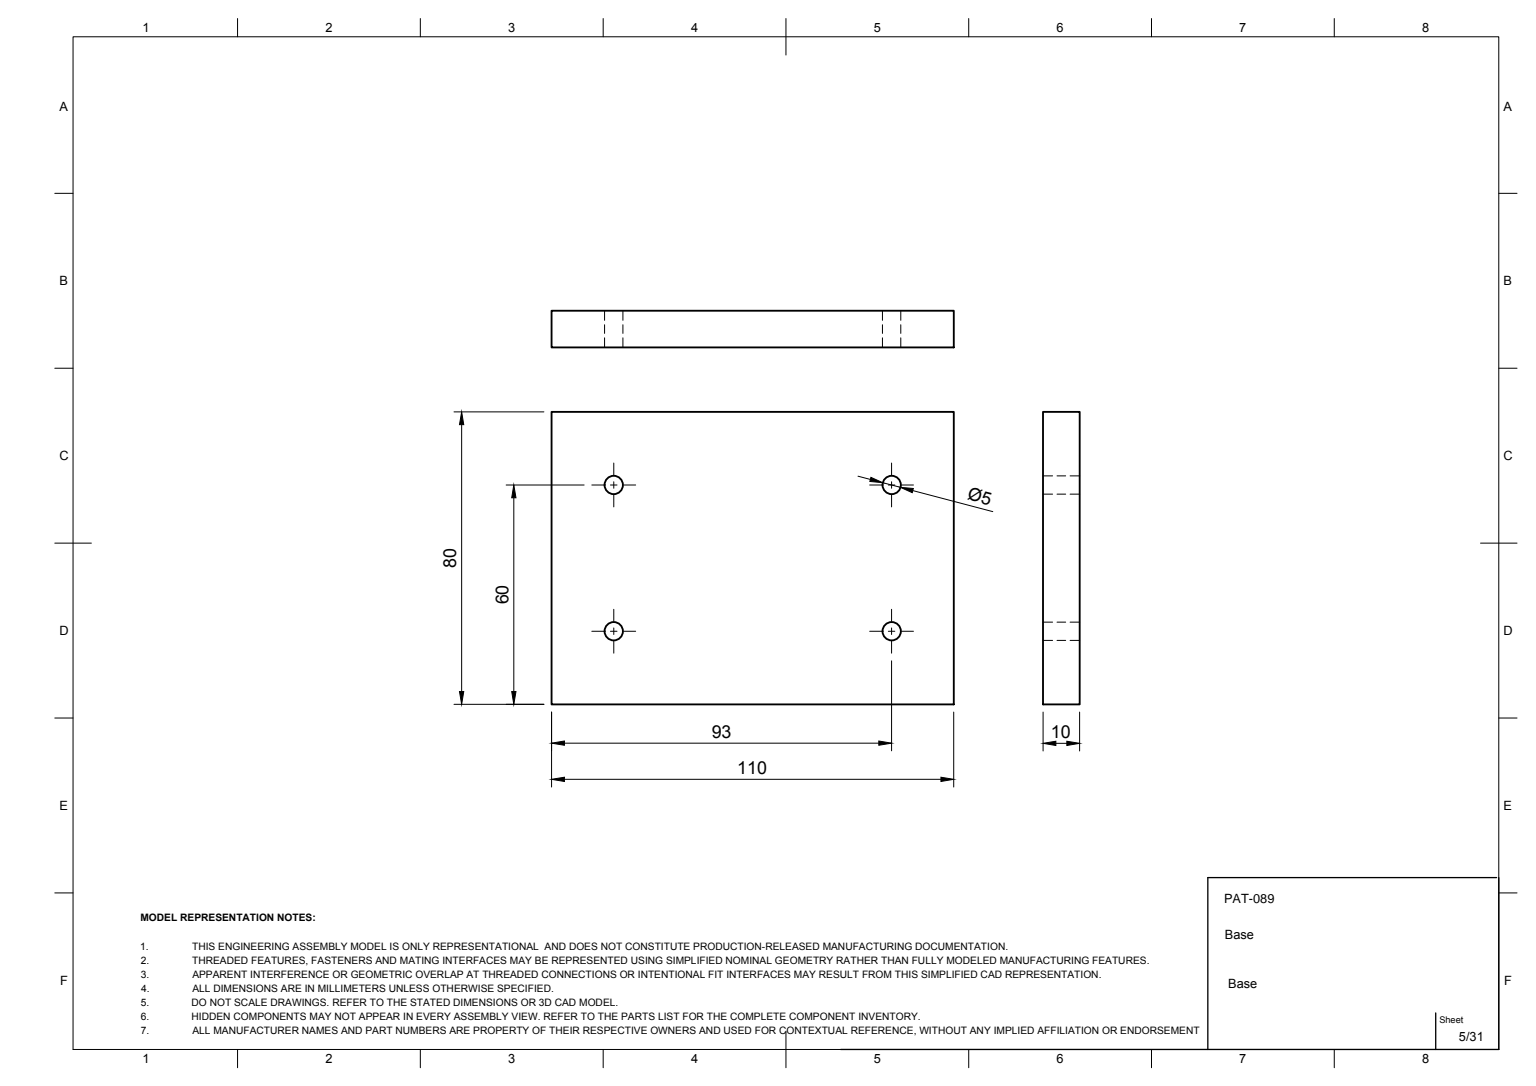
ISO-10303-21;
HEADER;
/* Generated by software containing ST-Developer
 * from STEP Tools, Inc. (www.steptools.com) 
 */

FILE_DESCRIPTION(
/* description */ ('Rotary union on bearing shaft'),
/* implementation_level */ '2;1');

FILE_NAME(
/* name */ 'Base.step',
/* time_stamp */ '2026-10-28T03:24:01-07:00',
/* author */ (''),
/* organization */ (''),
/* preprocessor_version */ 'ST-DEVELOPER v20.2',
/* originating_system */ 'Autodesk Translation Framework v15.17.0.0',
/* authorisation */ '');

FILE_SCHEMA (('AUTOMOTIVE_DESIGN { 1 0 10303 214 3 1 1 }'));
ENDSEC;

DATA;
#10=MECHANICAL_DESIGN_GEOMETRIC_PRESENTATION_REPRESENTATION('',(#313),#9448);
#259=SHAPE_REPRESENTATION_RELATIONSHIP('SRR','None',#9559,#286);
#286=ADVANCED_BREP_SHAPE_REPRESENTATION('',(#348),#9419);
#313=STYLED_ITEM('',(#9757),#348);
#348=MANIFOLD_SOLID_BREP('Body1',#4868);
#380=FACE_BOUND('',#964,.T.);
#381=FACE_BOUND('',#965,.T.);
#382=FACE_BOUND('',#966,.T.);
#383=FACE_BOUND('',#967,.T.);
#384=FACE_BOUND('',#969,.T.);
#385=FACE_BOUND('',#970,.T.);
#386=FACE_BOUND('',#971,.T.);
#387=FACE_BOUND('',#972,.T.);
#487=PLANE('',#5219);
#488=PLANE('',#5220);
#489=PLANE('',#5221);
#490=PLANE('',#5222);
#491=PLANE('',#5223);
#492=PLANE('',#5224);
#656=FACE_OUTER_BOUND('',#955,.T.);
#657=FACE_OUTER_BOUND('',#956,.T.);
#658=FACE_OUTER_BOUND('',#957,.T.);
#659=FACE_OUTER_BOUND('',#958,.T.);
#660=FACE_OUTER_BOUND('',#959,.T.);
#661=FACE_OUTER_BOUND('',#960,.T.);
#662=FACE_OUTER_BOUND('',#961,.T.);
#663=FACE_OUTER_BOUND('',#962,.T.);
#664=FACE_OUTER_BOUND('',#963,.T.);
#665=FACE_OUTER_BOUND('',#968,.T.);
#955=EDGE_LOOP('',(#3267,#3268,#3269,#3270));
#956=EDGE_LOOP('',(#3271,#3272,#3273,#3274));
#957=EDGE_LOOP('',(#3275,#3276,#3277,#3278));
#958=EDGE_LOOP('',(#3279,#3280,#3281,#3282));
#959=EDGE_LOOP('',(#3283,#3284,#3285,#3286));
#960=EDGE_LOOP('',(#3287,#3288,#3289,#3290));
#961=EDGE_LOOP('',(#3291,#3292,#3293,#3294));
#962=EDGE_LOOP('',(#3295,#3296,#3297,#3298));
#963=EDGE_LOOP('',(#3299,#3300,#3301,#3302));
#964=EDGE_LOOP('',(#3303));
#965=EDGE_LOOP('',(#3304));
#966=EDGE_LOOP('',(#3305));
#967=EDGE_LOOP('',(#3306));
#968=EDGE_LOOP('',(#3307,#3308,#3309,#3310));
#969=EDGE_LOOP('',(#3311));
#970=EDGE_LOOP('',(#3312));
#971=EDGE_LOOP('',(#3313));
#972=EDGE_LOOP('',(#3314));
#1361=LINE('',#7403,#1681);
#1362=LINE('',#7409,#1682);
#1363=LINE('',#7415,#1683);
#1364=LINE('',#7421,#1684);
#1365=LINE('',#7426,#1685);
#1366=LINE('',#7428,#1686);
#1367=LINE('',#7430,#1687);
#1368=LINE('',#7431,#1688);
#1369=LINE('',#7434,#1689);
#1370=LINE('',#7436,#1690);
#1371=LINE('',#7437,#1691);
#1372=LINE('',#7440,#1692);
#1373=LINE('',#7442,#1693);
#1374=LINE('',#7443,#1694);
#1375=LINE('',#7445,#1695);
#1376=LINE('',#7446,#1696);
#1681=VECTOR('',#5838,0.25);
#1682=VECTOR('',#5845,0.25);
#1683=VECTOR('',#5852,0.25);
#1684=VECTOR('',#5859,0.25);
#1685=VECTOR('',#5864,1.);
#1686=VECTOR('',#5865,1.);
#1687=VECTOR('',#5866,1.);
#1688=VECTOR('',#5867,1.);
#1689=VECTOR('',#5870,1.);
#1690=VECTOR('',#5871,1.);
#1691=VECTOR('',#5872,1.);
#1692=VECTOR('',#5875,1.);
#1693=VECTOR('',#5876,1.);
#1694=VECTOR('',#5877,1.);
#1695=VECTOR('',#5880,1.);
#1696=VECTOR('',#5881,1.);
#2001=CIRCLE('',#5208,0.25);
#2002=CIRCLE('',#5209,0.25);
#2003=CIRCLE('',#5211,0.25);
#2004=CIRCLE('',#5212,0.25);
#2005=CIRCLE('',#5214,0.25);
#2006=CIRCLE('',#5215,0.25);
#2007=CIRCLE('',#5217,0.25);
#2008=CIRCLE('',#5218,0.25);
#2253=VERTEX_POINT('',#7400);
#2254=VERTEX_POINT('',#7402);
#2255=VERTEX_POINT('',#7406);
#2256=VERTEX_POINT('',#7408);
#2257=VERTEX_POINT('',#7412);
#2258=VERTEX_POINT('',#7414);
#2259=VERTEX_POINT('',#7418);
#2260=VERTEX_POINT('',#7420);
#2261=VERTEX_POINT('',#7424);
#2262=VERTEX_POINT('',#7425);
#2263=VERTEX_POINT('',#7427);
#2264=VERTEX_POINT('',#7429);
#2265=VERTEX_POINT('',#7433);
#2266=VERTEX_POINT('',#7435);
#2267=VERTEX_POINT('',#7439);
#2268=VERTEX_POINT('',#7441);
#2661=EDGE_CURVE('',#2253,#2253,#2001,.T.);
#2662=EDGE_CURVE('',#2253,#2254,#1361,.T.);
#2663=EDGE_CURVE('',#2254,#2254,#2002,.T.);
#2664=EDGE_CURVE('',#2255,#2255,#2003,.T.);
#2665=EDGE_CURVE('',#2255,#2256,#1362,.T.);
#2666=EDGE_CURVE('',#2256,#2256,#2004,.T.);
#2667=EDGE_CURVE('',#2257,#2257,#2005,.T.);
#2668=EDGE_CURVE('',#2257,#2258,#1363,.T.);
#2669=EDGE_CURVE('',#2258,#2258,#2006,.T.);
#2670=EDGE_CURVE('',#2259,#2259,#2007,.T.);
#2671=EDGE_CURVE('',#2259,#2260,#1364,.T.);
#2672=EDGE_CURVE('',#2260,#2260,#2008,.T.);
#2673=EDGE_CURVE('',#2261,#2262,#1365,.T.);
#2674=EDGE_CURVE('',#2262,#2263,#1366,.T.);
#2675=EDGE_CURVE('',#2264,#2263,#1367,.T.);
#2676=EDGE_CURVE('',#2261,#2264,#1368,.T.);
#2677=EDGE_CURVE('',#2265,#2261,#1369,.T.);
#2678=EDGE_CURVE('',#2266,#2264,#1370,.T.);
#2679=EDGE_CURVE('',#2265,#2266,#1371,.T.);
#2680=EDGE_CURVE('',#2267,#2265,#1372,.T.);
#2681=EDGE_CURVE('',#2268,#2266,#1373,.T.);
#2682=EDGE_CURVE('',#2267,#2268,#1374,.T.);
#2683=EDGE_CURVE('',#2262,#2267,#1375,.T.);
#2684=EDGE_CURVE('',#2263,#2268,#1376,.T.);
#3267=ORIENTED_EDGE('',*,*,#2661,.F.);
#3268=ORIENTED_EDGE('',*,*,#2662,.T.);
#3269=ORIENTED_EDGE('',*,*,#2663,.F.);
#3270=ORIENTED_EDGE('',*,*,#2662,.F.);
#3271=ORIENTED_EDGE('',*,*,#2664,.F.);
#3272=ORIENTED_EDGE('',*,*,#2665,.T.);
#3273=ORIENTED_EDGE('',*,*,#2666,.F.);
#3274=ORIENTED_EDGE('',*,*,#2665,.F.);
#3275=ORIENTED_EDGE('',*,*,#2667,.F.);
#3276=ORIENTED_EDGE('',*,*,#2668,.T.);
#3277=ORIENTED_EDGE('',*,*,#2669,.F.);
#3278=ORIENTED_EDGE('',*,*,#2668,.F.);
#3279=ORIENTED_EDGE('',*,*,#2670,.F.);
#3280=ORIENTED_EDGE('',*,*,#2671,.T.);
#3281=ORIENTED_EDGE('',*,*,#2672,.F.);
#3282=ORIENTED_EDGE('',*,*,#2671,.F.);
#3283=ORIENTED_EDGE('',*,*,#2673,.T.);
#3284=ORIENTED_EDGE('',*,*,#2674,.T.);
#3285=ORIENTED_EDGE('',*,*,#2675,.F.);
#3286=ORIENTED_EDGE('',*,*,#2676,.F.);
#3287=ORIENTED_EDGE('',*,*,#2677,.T.);
#3288=ORIENTED_EDGE('',*,*,#2676,.T.);
#3289=ORIENTED_EDGE('',*,*,#2678,.F.);
#3290=ORIENTED_EDGE('',*,*,#2679,.F.);
#3291=ORIENTED_EDGE('',*,*,#2680,.T.);
#3292=ORIENTED_EDGE('',*,*,#2679,.T.);
#3293=ORIENTED_EDGE('',*,*,#2681,.F.);
#3294=ORIENTED_EDGE('',*,*,#2682,.F.);
#3295=ORIENTED_EDGE('',*,*,#2683,.T.);
#3296=ORIENTED_EDGE('',*,*,#2682,.T.);
#3297=ORIENTED_EDGE('',*,*,#2684,.F.);
#3298=ORIENTED_EDGE('',*,*,#2674,.F.);
#3299=ORIENTED_EDGE('',*,*,#2684,.T.);
#3300=ORIENTED_EDGE('',*,*,#2681,.T.);
#3301=ORIENTED_EDGE('',*,*,#2678,.T.);
#3302=ORIENTED_EDGE('',*,*,#2675,.T.);
#3303=ORIENTED_EDGE('',*,*,#2663,.T.);
#3304=ORIENTED_EDGE('',*,*,#2666,.T.);
#3305=ORIENTED_EDGE('',*,*,#2669,.T.);
#3306=ORIENTED_EDGE('',*,*,#2672,.T.);
#3307=ORIENTED_EDGE('',*,*,#2683,.F.);
#3308=ORIENTED_EDGE('',*,*,#2673,.F.);
#3309=ORIENTED_EDGE('',*,*,#2677,.F.);
#3310=ORIENTED_EDGE('',*,*,#2680,.F.);
#3311=ORIENTED_EDGE('',*,*,#2661,.T.);
#3312=ORIENTED_EDGE('',*,*,#2664,.T.);
#3313=ORIENTED_EDGE('',*,*,#2667,.T.);
#3314=ORIENTED_EDGE('',*,*,#2670,.T.);
#4479=CYLINDRICAL_SURFACE('',#5207,0.25);
#4480=CYLINDRICAL_SURFACE('',#5210,0.25);
#4481=CYLINDRICAL_SURFACE('',#5213,0.25);
#4482=CYLINDRICAL_SURFACE('',#5216,0.25);
#4569=ADVANCED_FACE('',(#656),#4479,.F.);
#4570=ADVANCED_FACE('',(#657),#4480,.F.);
#4571=ADVANCED_FACE('',(#658),#4481,.F.);
#4572=ADVANCED_FACE('',(#659),#4482,.F.);
#4573=ADVANCED_FACE('',(#660),#487,.T.);
#4574=ADVANCED_FACE('',(#661),#488,.T.);
#4575=ADVANCED_FACE('',(#662),#489,.T.);
#4576=ADVANCED_FACE('',(#663),#490,.T.);
#4577=ADVANCED_FACE('',(#664,#380,#381,#382,#383),#491,.T.);
#4578=ADVANCED_FACE('',(#665,#384,#385,#386,#387),#492,.F.);
#4868=CLOSED_SHELL('',(#4569,#4570,#4571,#4572,#4573,#4574,#4575,#4576,
#4577,#4578));
#5206=AXIS2_PLACEMENT_3D('',#7398,#5832,#5833);
#5207=AXIS2_PLACEMENT_3D('',#7399,#5834,#5835);
#5208=AXIS2_PLACEMENT_3D('',#7401,#5836,#5837);
#5209=AXIS2_PLACEMENT_3D('',#7404,#5839,#5840);
#5210=AXIS2_PLACEMENT_3D('',#7405,#5841,#5842);
#5211=AXIS2_PLACEMENT_3D('',#7407,#5843,#5844);
#5212=AXIS2_PLACEMENT_3D('',#7410,#5846,#5847);
#5213=AXIS2_PLACEMENT_3D('',#7411,#5848,#5849);
#5214=AXIS2_PLACEMENT_3D('',#7413,#5850,#5851);
#5215=AXIS2_PLACEMENT_3D('',#7416,#5853,#5854);
#5216=AXIS2_PLACEMENT_3D('',#7417,#5855,#5856);
#5217=AXIS2_PLACEMENT_3D('',#7419,#5857,#5858);
#5218=AXIS2_PLACEMENT_3D('',#7422,#5860,#5861);
#5219=AXIS2_PLACEMENT_3D('',#7423,#5862,#5863);
#5220=AXIS2_PLACEMENT_3D('',#7432,#5868,#5869);
#5221=AXIS2_PLACEMENT_3D('',#7438,#5873,#5874);
#5222=AXIS2_PLACEMENT_3D('',#7444,#5878,#5879);
#5223=AXIS2_PLACEMENT_3D('',#7447,#5882,#5883);
#5224=AXIS2_PLACEMENT_3D('',#7448,#5884,#5885);
#5832=DIRECTION('axis',(0.,0.,1.));
#5833=DIRECTION('refdir',(1.,0.,0.));
#5834=DIRECTION('center_axis',(0.,0.,1.));
#5835=DIRECTION('ref_axis',(1.,0.,0.));
#5836=DIRECTION('center_axis',(0.,0.,1.));
#5837=DIRECTION('ref_axis',(1.,0.,0.));
#5838=DIRECTION('',(0.,0.,1.));
#5839=DIRECTION('center_axis',(0.,0.,-1.));
#5840=DIRECTION('ref_axis',(1.,0.,0.));
#5841=DIRECTION('center_axis',(0.,0.,1.));
#5842=DIRECTION('ref_axis',(1.,0.,0.));
#5843=DIRECTION('center_axis',(0.,0.,1.));
#5844=DIRECTION('ref_axis',(1.,0.,0.));
#5845=DIRECTION('',(0.,0.,1.));
#5846=DIRECTION('center_axis',(0.,0.,-1.));
#5847=DIRECTION('ref_axis',(1.,0.,0.));
#5848=DIRECTION('center_axis',(0.,0.,1.));
#5849=DIRECTION('ref_axis',(1.,0.,0.));
#5850=DIRECTION('center_axis',(0.,0.,1.));
#5851=DIRECTION('ref_axis',(1.,0.,0.));
#5852=DIRECTION('',(0.,0.,1.));
#5853=DIRECTION('center_axis',(0.,0.,-1.));
#5854=DIRECTION('ref_axis',(1.,0.,0.));
#5855=DIRECTION('center_axis',(0.,0.,1.));
#5856=DIRECTION('ref_axis',(1.,0.,0.));
#5857=DIRECTION('center_axis',(0.,0.,1.));
#5858=DIRECTION('ref_axis',(1.,0.,0.));
#5859=DIRECTION('',(0.,0.,1.));
#5860=DIRECTION('center_axis',(0.,0.,-1.));
#5861=DIRECTION('ref_axis',(1.,0.,0.));
#5862=DIRECTION('center_axis',(0.,1.,0.));
#5863=DIRECTION('ref_axis',(-1.,0.,0.));
#5864=DIRECTION('',(-1.,0.,0.));
#5865=DIRECTION('',(0.,0.,1.));
#5866=DIRECTION('',(-1.,0.,0.));
#5867=DIRECTION('',(0.,0.,1.));
#5868=DIRECTION('center_axis',(1.,0.,0.));
#5869=DIRECTION('ref_axis',(0.,1.,0.));
#5870=DIRECTION('',(0.,1.,0.));
#5871=DIRECTION('',(0.,1.,0.));
#5872=DIRECTION('',(0.,0.,1.));
#5873=DIRECTION('center_axis',(0.,-1.,0.));
#5874=DIRECTION('ref_axis',(1.,0.,0.));
#5875=DIRECTION('',(1.,0.,0.));
#5876=DIRECTION('',(1.,0.,0.));
#5877=DIRECTION('',(0.,0.,1.));
#5878=DIRECTION('center_axis',(-1.,0.,0.));
#5879=DIRECTION('ref_axis',(0.,-1.,0.));
#5880=DIRECTION('',(0.,-1.,0.));
#5881=DIRECTION('',(0.,-1.,0.));
#5882=DIRECTION('center_axis',(0.,0.,1.));
#5883=DIRECTION('ref_axis',(1.,0.,0.));
#5884=DIRECTION('center_axis',(0.,0.,1.));
#5885=DIRECTION('ref_axis',(1.,0.,0.));
#7398=CARTESIAN_POINT('',(0.,0.,0.));
#7399=CARTESIAN_POINT('Origin',(3.8,1.,-0.1));
#7400=CARTESIAN_POINT('',(3.55,1.,0.));
#7401=CARTESIAN_POINT('Origin',(3.8,1.,0.));
#7402=CARTESIAN_POINT('',(3.55,1.,1.));
#7403=CARTESIAN_POINT('',(3.55,1.,-0.1));
#7404=CARTESIAN_POINT('Origin',(3.8,1.,1.));
#7405=CARTESIAN_POINT('Origin',(-3.8,5.,-0.1));
#7406=CARTESIAN_POINT('',(-4.05,5.,0.));
#7407=CARTESIAN_POINT('Origin',(-3.8,5.,0.));
#7408=CARTESIAN_POINT('',(-4.05,5.,1.));
#7409=CARTESIAN_POINT('',(-4.05,5.,-0.1));
#7410=CARTESIAN_POINT('Origin',(-3.8,5.,1.));
#7411=CARTESIAN_POINT('Origin',(-3.8,1.,-0.1));
#7412=CARTESIAN_POINT('',(-4.05,1.,0.));
#7413=CARTESIAN_POINT('Origin',(-3.8,1.,0.));
#7414=CARTESIAN_POINT('',(-4.05,1.,1.));
#7415=CARTESIAN_POINT('',(-4.05,1.,-0.1));
#7416=CARTESIAN_POINT('Origin',(-3.8,1.,1.));
#7417=CARTESIAN_POINT('Origin',(3.8,5.,-0.1));
#7418=CARTESIAN_POINT('',(3.55,5.,0.));
#7419=CARTESIAN_POINT('Origin',(3.8,5.,0.));
#7420=CARTESIAN_POINT('',(3.55,5.,1.));
#7421=CARTESIAN_POINT('',(3.55,5.,-0.1));
#7422=CARTESIAN_POINT('Origin',(3.8,5.,1.));
#7423=CARTESIAN_POINT('Origin',(5.5,7.,0.));
#7424=CARTESIAN_POINT('',(5.5,7.,0.));
#7425=CARTESIAN_POINT('',(-5.5,7.,0.));
#7426=CARTESIAN_POINT('',(5.5,7.,0.));
#7427=CARTESIAN_POINT('',(-5.5,7.,1.));
#7428=CARTESIAN_POINT('',(-5.5,7.,0.));
#7429=CARTESIAN_POINT('',(5.5,7.,1.));
#7430=CARTESIAN_POINT('',(5.5,7.,1.));
#7431=CARTESIAN_POINT('',(5.5,7.,0.));
#7432=CARTESIAN_POINT('Origin',(5.5,-1.,0.));
#7433=CARTESIAN_POINT('',(5.5,-1.,0.));
#7434=CARTESIAN_POINT('',(5.5,-1.,0.));
#7435=CARTESIAN_POINT('',(5.5,-1.,1.));
#7436=CARTESIAN_POINT('',(5.5,-1.,1.));
#7437=CARTESIAN_POINT('',(5.5,-1.,0.));
#7438=CARTESIAN_POINT('Origin',(-5.5,-1.,0.));
#7439=CARTESIAN_POINT('',(-5.5,-1.,0.));
#7440=CARTESIAN_POINT('',(-5.5,-1.,0.));
#7441=CARTESIAN_POINT('',(-5.5,-1.,1.));
#7442=CARTESIAN_POINT('',(-5.5,-1.,1.));
#7443=CARTESIAN_POINT('',(-5.5,-1.,0.));
#7444=CARTESIAN_POINT('Origin',(-5.5,7.,0.));
#7445=CARTESIAN_POINT('',(-5.5,7.,0.));
#7446=CARTESIAN_POINT('',(-5.5,7.,1.));
#7447=CARTESIAN_POINT('Origin',(0.,3.,1.));
#7448=CARTESIAN_POINT('Origin',(0.,3.,0.));
#9387=UNCERTAINTY_MEASURE_WITH_UNIT(LENGTH_MEASURE(0.001),#9449,
'DISTANCE_ACCURACY_VALUE',
'Maximum model space distance between geometric entities at asserted c
onnectivities');
#9416=UNCERTAINTY_MEASURE_WITH_UNIT(LENGTH_MEASURE(0.001),#9449,
'DISTANCE_ACCURACY_VALUE',
'Maximum model space distance between geometric entities at asserted c
onnectivities');
#9419=(
GEOMETRIC_REPRESENTATION_CONTEXT(3)
GLOBAL_UNCERTAINTY_ASSIGNED_CONTEXT((#9387))
GLOBAL_UNIT_ASSIGNED_CONTEXT((#9449,#9451,#9452))
REPRESENTATION_CONTEXT('','3D')
);
#9448=(
GEOMETRIC_REPRESENTATION_CONTEXT(3)
GLOBAL_UNCERTAINTY_ASSIGNED_CONTEXT((#9416))
GLOBAL_UNIT_ASSIGNED_CONTEXT((#9449,#9451,#9452))
REPRESENTATION_CONTEXT('','3D')
);
#9449=(
LENGTH_UNIT()
NAMED_UNIT(*)
SI_UNIT(.CENTI.,.METRE.)
);
#9451=(
NAMED_UNIT(*)
PLANE_ANGLE_UNIT()
SI_UNIT($,.RADIAN.)
);
#9452=(
NAMED_UNIT(*)
SI_UNIT($,.STERADIAN.)
SOLID_ANGLE_UNIT()
);
#9455=SHAPE_DEFINITION_REPRESENTATION(#9486,#9559);
#9486=PRODUCT_DEFINITION_SHAPE('',$,#9591);
#9559=SHAPE_REPRESENTATION('',(#5206),#9419);
#9588=PRODUCT_DEFINITION_CONTEXT('part definition',#9683,'design');
#9591=PRODUCT_DEFINITION('Base','Base',#9622,#9588);
#9622=PRODUCT_DEFINITION_FORMATION('',$,#9687);
#9683=APPLICATION_CONTEXT(
'Core Data for Automotive Mechanical Design Process');
#9684=PRODUCT_CONTEXT('part definition',#9683,'mechanical');
#9687=PRODUCT('Base','Base','Base',(#9684));
#9751=COLOUR_RGB('Dark Blue',0.08,0.2,0.34);
#9752=FILL_AREA_STYLE_COLOUR('',#9751);
#9753=FILL_AREA_STYLE('',(#9752));
#9754=SURFACE_STYLE_FILL_AREA(#9753);
#9755=SURFACE_SIDE_STYLE('',(#9754));
#9756=SURFACE_STYLE_USAGE(.BOTH.,#9755);
#9757=PRESENTATION_STYLE_ASSIGNMENT((#9756));
ENDSEC;
END-ISO-10303-21;
